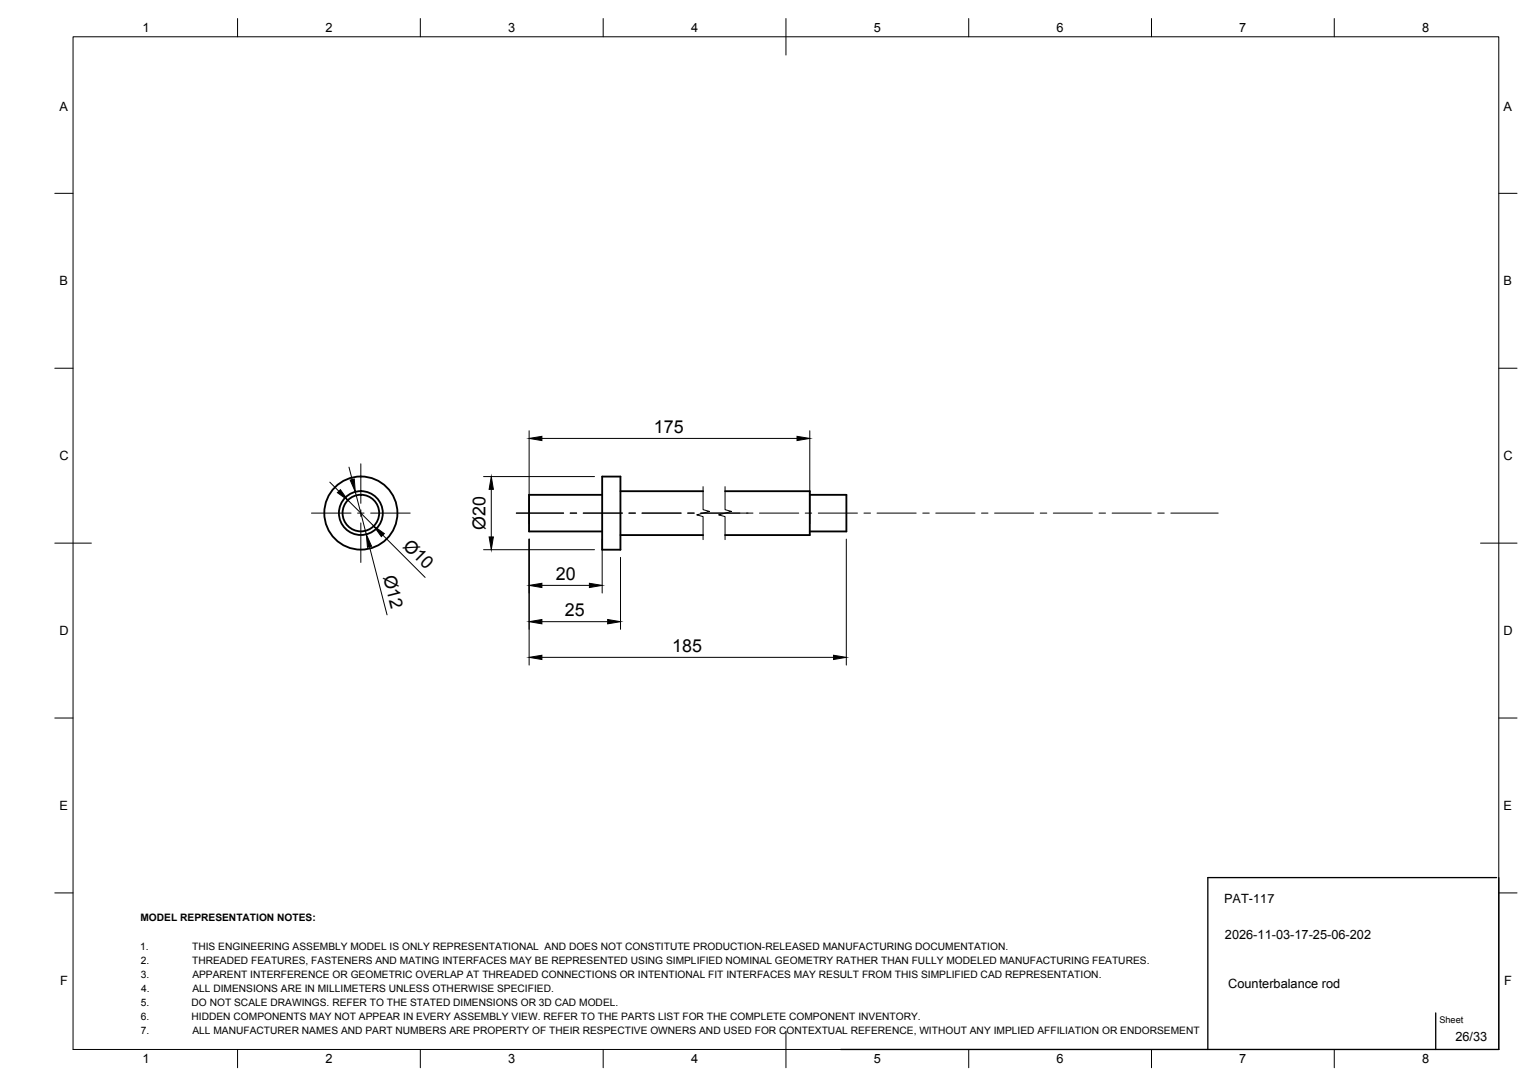
ISO-10303-21;
HEADER;
/* Generated by software containing ST-Developer
 * from STEP Tools, Inc. (www.steptools.com) 
 */

FILE_DESCRIPTION(
/* description */ ('Counterbalanced vertical column'),
/* implementation_level */ '2;1');

FILE_NAME(
/* name */ 'Counterbalance rod.step',
/* time_stamp */ '2026-10-29T16:47:22-07:00',
/* author */ (''),
/* organization */ (''),
/* preprocessor_version */ 'ST-DEVELOPER v20.2',
/* originating_system */ 'Autodesk Translation Framework v15.17.0.0',
/* authorisation */ '');

FILE_SCHEMA (('AUTOMOTIVE_DESIGN { 1 0 10303 214 3 1 1 }'));
ENDSEC;

DATA;
#10=MECHANICAL_DESIGN_GEOMETRIC_PRESENTATION_REPRESENTATION('',(#375),#15040);
#305=SHAPE_REPRESENTATION_RELATIONSHIP('SRR','None',#15210,#340);
#340=ADVANCED_BREP_SHAPE_REPRESENTATION('',(#408),#15029);
#375=STYLED_ITEM('',(#15457),#408);
#408=MANIFOLD_SOLID_BREP('Body1',#7100);
#516=FACE_BOUND('',#1633,.T.);
#517=FACE_BOUND('',#1636,.T.);
#518=FACE_BOUND('',#1639,.T.);
#743=PLANE('',#7996);
#744=PLANE('',#8000);
#745=PLANE('',#8001);
#746=PLANE('',#8006);
#747=PLANE('',#8009);
#1123=FACE_OUTER_BOUND('',#1628,.T.);
#1124=FACE_OUTER_BOUND('',#1629,.T.);
#1125=FACE_OUTER_BOUND('',#1630,.T.);
#1126=FACE_OUTER_BOUND('',#1631,.T.);
#1127=FACE_OUTER_BOUND('',#1632,.T.);
#1128=FACE_OUTER_BOUND('',#1634,.T.);
#1129=FACE_OUTER_BOUND('',#1635,.T.);
#1130=FACE_OUTER_BOUND('',#1637,.T.);
#1131=FACE_OUTER_BOUND('',#1638,.T.);
#1628=EDGE_LOOP('',(#6102,#6103,#6104,#6105));
#1629=EDGE_LOOP('',(#6106));
#1630=EDGE_LOOP('',(#6107,#6108,#6109,#6110));
#1631=EDGE_LOOP('',(#6111));
#1632=EDGE_LOOP('',(#6112));
#1633=EDGE_LOOP('',(#6113));
#1634=EDGE_LOOP('',(#6114,#6115,#6116,#6117));
#1635=EDGE_LOOP('',(#6118));
#1636=EDGE_LOOP('',(#6119));
#1637=EDGE_LOOP('',(#6120,#6121,#6122,#6123));
#1638=EDGE_LOOP('',(#6124));
#1639=EDGE_LOOP('',(#6125));
#2237=LINE('',#14397,#2908);
#2238=LINE('',#14404,#2909);
#2239=LINE('',#14415,#2910);
#2240=LINE('',#14419,#2911);
#2908=VECTOR('',#9701,0.5);
#2909=VECTOR('',#9710,0.5);
#2910=VECTOR('',#9725,1.);
#2911=VECTOR('',#9730,0.6);
#3255=CIRCLE('',#7994,0.5);
#3256=CIRCLE('',#7995,0.5);
#3257=CIRCLE('',#7998,0.5);
#3258=CIRCLE('',#7999,0.5);
#3259=CIRCLE('',#8002,1.);
#3260=CIRCLE('',#8003,0.6);
#3261=CIRCLE('',#8005,1.);
#3262=CIRCLE('',#8008,0.6);
#3740=VERTEX_POINT('',#14394);
#3741=VERTEX_POINT('',#14396);
#3742=VERTEX_POINT('',#14401);
#3743=VERTEX_POINT('',#14403);
#3744=VERTEX_POINT('',#14408);
#3745=VERTEX_POINT('',#14410);
#3746=VERTEX_POINT('',#14413);
#3747=VERTEX_POINT('',#14418);
#4552=EDGE_CURVE('',#3740,#3740,#3255,.T.);
#4553=EDGE_CURVE('',#3740,#3741,#2237,.T.);
#4554=EDGE_CURVE('',#3741,#3741,#3256,.T.);
#4555=EDGE_CURVE('',#3742,#3742,#3257,.T.);
#4556=EDGE_CURVE('',#3742,#3743,#2238,.T.);
#4557=EDGE_CURVE('',#3743,#3743,#3258,.T.);
#4558=EDGE_CURVE('',#3744,#3744,#3259,.T.);
#4559=EDGE_CURVE('',#3745,#3745,#3260,.T.);
#4560=EDGE_CURVE('',#3746,#3746,#3261,.T.);
#4561=EDGE_CURVE('',#3746,#3744,#2239,.T.);
#4562=EDGE_CURVE('',#3745,#3747,#2240,.T.);
#4563=EDGE_CURVE('',#3747,#3747,#3262,.T.);
#6102=ORIENTED_EDGE('',*,*,#4552,.F.);
#6103=ORIENTED_EDGE('',*,*,#4553,.T.);
#6104=ORIENTED_EDGE('',*,*,#4554,.F.);
#6105=ORIENTED_EDGE('',*,*,#4553,.F.);
#6106=ORIENTED_EDGE('',*,*,#4552,.T.);
#6107=ORIENTED_EDGE('',*,*,#4555,.F.);
#6108=ORIENTED_EDGE('',*,*,#4556,.T.);
#6109=ORIENTED_EDGE('',*,*,#4557,.T.);
#6110=ORIENTED_EDGE('',*,*,#4556,.F.);
#6111=ORIENTED_EDGE('',*,*,#4557,.F.);
#6112=ORIENTED_EDGE('',*,*,#4558,.F.);
#6113=ORIENTED_EDGE('',*,*,#4559,.T.);
#6114=ORIENTED_EDGE('',*,*,#4560,.F.);
#6115=ORIENTED_EDGE('',*,*,#4561,.T.);
#6116=ORIENTED_EDGE('',*,*,#4558,.T.);
#6117=ORIENTED_EDGE('',*,*,#4561,.F.);
#6118=ORIENTED_EDGE('',*,*,#4560,.T.);
#6119=ORIENTED_EDGE('',*,*,#4554,.T.);
#6120=ORIENTED_EDGE('',*,*,#4559,.F.);
#6121=ORIENTED_EDGE('',*,*,#4562,.T.);
#6122=ORIENTED_EDGE('',*,*,#4563,.T.);
#6123=ORIENTED_EDGE('',*,*,#4562,.F.);
#6124=ORIENTED_EDGE('',*,*,#4563,.F.);
#6125=ORIENTED_EDGE('',*,*,#4555,.T.);
#6650=CYLINDRICAL_SURFACE('',#7993,0.5);
#6651=CYLINDRICAL_SURFACE('',#7997,0.5);
#6652=CYLINDRICAL_SURFACE('',#8004,1.);
#6653=CYLINDRICAL_SURFACE('',#8007,0.6);
#6965=ADVANCED_FACE('',(#1123),#6650,.T.);
#6966=ADVANCED_FACE('',(#1124),#743,.T.);
#6967=ADVANCED_FACE('',(#1125),#6651,.T.);
#6968=ADVANCED_FACE('',(#1126),#744,.F.);
#6969=ADVANCED_FACE('',(#1127,#516),#745,.F.);
#6970=ADVANCED_FACE('',(#1128),#6652,.T.);
#6971=ADVANCED_FACE('',(#1129,#517),#746,.T.);
#6972=ADVANCED_FACE('',(#1130),#6653,.T.);
#6973=ADVANCED_FACE('',(#1131,#518),#747,.F.);
#7100=CLOSED_SHELL('',(#6965,#6966,#6967,#6968,#6969,#6970,#6971,#6972,
#6973));
#7992=AXIS2_PLACEMENT_3D('',#14392,#9695,#9696);
#7993=AXIS2_PLACEMENT_3D('',#14393,#9697,#9698);
#7994=AXIS2_PLACEMENT_3D('',#14395,#9699,#9700);
#7995=AXIS2_PLACEMENT_3D('',#14398,#9702,#9703);
#7996=AXIS2_PLACEMENT_3D('',#14399,#9704,#9705);
#7997=AXIS2_PLACEMENT_3D('',#14400,#9706,#9707);
#7998=AXIS2_PLACEMENT_3D('',#14402,#9708,#9709);
#7999=AXIS2_PLACEMENT_3D('',#14405,#9711,#9712);
#8000=AXIS2_PLACEMENT_3D('',#14406,#9713,#9714);
#8001=AXIS2_PLACEMENT_3D('',#14407,#9715,#9716);
#8002=AXIS2_PLACEMENT_3D('',#14409,#9717,#9718);
#8003=AXIS2_PLACEMENT_3D('',#14411,#9719,#9720);
#8004=AXIS2_PLACEMENT_3D('',#14412,#9721,#9722);
#8005=AXIS2_PLACEMENT_3D('',#14414,#9723,#9724);
#8006=AXIS2_PLACEMENT_3D('',#14416,#9726,#9727);
#8007=AXIS2_PLACEMENT_3D('',#14417,#9728,#9729);
#8008=AXIS2_PLACEMENT_3D('',#14420,#9731,#9732);
#8009=AXIS2_PLACEMENT_3D('',#14421,#9733,#9734);
#9695=DIRECTION('axis',(0.,0.,1.));
#9696=DIRECTION('refdir',(1.,0.,0.));
#9697=DIRECTION('center_axis',(0.,0.,1.));
#9698=DIRECTION('ref_axis',(1.,0.,0.));
#9699=DIRECTION('center_axis',(0.,0.,1.));
#9700=DIRECTION('ref_axis',(1.,0.,0.));
#9701=DIRECTION('',(0.,0.,-1.));
#9702=DIRECTION('center_axis',(0.,0.,-1.));
#9703=DIRECTION('ref_axis',(1.,0.,0.));
#9704=DIRECTION('center_axis',(0.,0.,1.));
#9705=DIRECTION('ref_axis',(1.,0.,0.));
#9706=DIRECTION('center_axis',(0.,0.,1.));
#9707=DIRECTION('ref_axis',(1.,0.,0.));
#9708=DIRECTION('center_axis',(0.,0.,1.));
#9709=DIRECTION('ref_axis',(1.,0.,0.));
#9710=DIRECTION('',(0.,0.,-1.));
#9711=DIRECTION('center_axis',(0.,0.,1.));
#9712=DIRECTION('ref_axis',(1.,0.,0.));
#9713=DIRECTION('center_axis',(0.,0.,1.));
#9714=DIRECTION('ref_axis',(1.,0.,0.));
#9715=DIRECTION('center_axis',(0.,0.,1.));
#9716=DIRECTION('ref_axis',(1.,0.,0.));
#9717=DIRECTION('center_axis',(0.,0.,1.));
#9718=DIRECTION('ref_axis',(1.,0.,0.));
#9719=DIRECTION('center_axis',(0.,0.,1.));
#9720=DIRECTION('ref_axis',(1.,0.,0.));
#9721=DIRECTION('center_axis',(0.,0.,1.));
#9722=DIRECTION('ref_axis',(1.,0.,0.));
#9723=DIRECTION('center_axis',(0.,0.,1.));
#9724=DIRECTION('ref_axis',(1.,0.,0.));
#9725=DIRECTION('',(0.,0.,-1.));
#9726=DIRECTION('center_axis',(0.,0.,1.));
#9727=DIRECTION('ref_axis',(1.,0.,0.));
#9728=DIRECTION('center_axis',(0.,0.,1.));
#9729=DIRECTION('ref_axis',(1.,0.,0.));
#9730=DIRECTION('',(0.,0.,-1.));
#9731=DIRECTION('center_axis',(0.,0.,1.));
#9732=DIRECTION('ref_axis',(1.,0.,0.));
#9733=DIRECTION('center_axis',(0.,0.,1.));
#9734=DIRECTION('ref_axis',(1.,0.,0.));
#14392=CARTESIAN_POINT('',(0.,0.,0.));
#14393=CARTESIAN_POINT('Origin',(-7.,0.,21.));
#14394=CARTESIAN_POINT('',(-7.5,-6.12323399573677E-17,23.));
#14395=CARTESIAN_POINT('Origin',(-7.,0.,23.));
#14396=CARTESIAN_POINT('',(-7.5,-6.12323399573677E-17,21.));
#14397=CARTESIAN_POINT('',(-7.5,-6.12323399573677E-17,21.));
#14398=CARTESIAN_POINT('Origin',(-7.,0.,21.));
#14399=CARTESIAN_POINT('Origin',(-7.,0.,23.));
#14400=CARTESIAN_POINT('Origin',(-7.,0.,4.5));
#14401=CARTESIAN_POINT('',(-7.5,-6.12323399573677E-17,5.5));
#14402=CARTESIAN_POINT('Origin',(-7.,0.,5.5));
#14403=CARTESIAN_POINT('',(-7.5,-6.12323399573677E-17,4.5));
#14404=CARTESIAN_POINT('',(-7.5,-6.12323399573677E-17,4.5));
#14405=CARTESIAN_POINT('Origin',(-7.,0.,4.5));
#14406=CARTESIAN_POINT('Origin',(-7.,0.,4.5));
#14407=CARTESIAN_POINT('Origin',(-7.,0.,20.5));
#14408=CARTESIAN_POINT('',(-8.,-1.22464679914735E-16,20.5));
#14409=CARTESIAN_POINT('Origin',(-7.,0.,20.5));
#14410=CARTESIAN_POINT('',(-7.6,-7.34788079488412E-17,20.5));
#14411=CARTESIAN_POINT('Origin',(-7.,0.,20.5));
#14412=CARTESIAN_POINT('Origin',(-7.,0.,20.5));
#14413=CARTESIAN_POINT('',(-8.,-1.22464679914735E-16,21.));
#14414=CARTESIAN_POINT('Origin',(-7.,0.,21.));
#14415=CARTESIAN_POINT('',(-8.,-1.22464679914735E-16,20.5));
#14416=CARTESIAN_POINT('Origin',(-7.,0.,21.));
#14417=CARTESIAN_POINT('Origin',(-7.,0.,5.5));
#14418=CARTESIAN_POINT('',(-7.6,-7.34788079488412E-17,5.5));
#14419=CARTESIAN_POINT('',(-7.6,-7.34788079488412E-17,5.5));
#14420=CARTESIAN_POINT('Origin',(-7.,0.,5.5));
#14421=CARTESIAN_POINT('Origin',(-7.,0.,5.5));
#14989=UNCERTAINTY_MEASURE_WITH_UNIT(LENGTH_MEASURE(0.001),#15041,
'DISTANCE_ACCURACY_VALUE',
'Maximum model space distance between geometric entities at asserted c
onnectivities');
#15000=UNCERTAINTY_MEASURE_WITH_UNIT(LENGTH_MEASURE(0.001),#15041,
'DISTANCE_ACCURACY_VALUE',
'Maximum model space distance between geometric entities at asserted c
onnectivities');
#15029=(
GEOMETRIC_REPRESENTATION_CONTEXT(3)
GLOBAL_UNCERTAINTY_ASSIGNED_CONTEXT((#14989))
GLOBAL_UNIT_ASSIGNED_CONTEXT((#15041,#15043,#15044))
REPRESENTATION_CONTEXT('','3D')
);
#15040=(
GEOMETRIC_REPRESENTATION_CONTEXT(3)
GLOBAL_UNCERTAINTY_ASSIGNED_CONTEXT((#15000))
GLOBAL_UNIT_ASSIGNED_CONTEXT((#15041,#15043,#15044))
REPRESENTATION_CONTEXT('','3D')
);
#15041=(
LENGTH_UNIT()
NAMED_UNIT(*)
SI_UNIT(.CENTI.,.METRE.)
);
#15043=(
NAMED_UNIT(*)
PLANE_ANGLE_UNIT()
SI_UNIT($,.RADIAN.)
);
#15044=(
NAMED_UNIT(*)
SI_UNIT($,.STERADIAN.)
SOLID_ANGLE_UNIT()
);
#15073=SHAPE_DEFINITION_REPRESENTATION(#15112,#15210);
#15112=PRODUCT_DEFINITION_SHAPE('',$,#15250);
#15210=SHAPE_REPRESENTATION('',(#7992),#15029);
#15221=PRODUCT_DEFINITION_CONTEXT('part definition',#15340,'design');
#15250=PRODUCT_DEFINITION('Counterbalance rod','Counterbalance rod',#15289,
#15221);
#15289=PRODUCT_DEFINITION_FORMATION('',$,#15370);
#15340=APPLICATION_CONTEXT(
'Core Data for Automotive Mechanical Design Process');
#15341=PRODUCT_CONTEXT('part definition',#15340,'mechanical');
#15370=PRODUCT('Counterbalance rod','Counterbalance rod',
'Counterbalance rod',(#15341));
#15451=COLOUR_RGB('Grey',0.48,0.52,0.57);
#15452=FILL_AREA_STYLE_COLOUR('',#15451);
#15453=FILL_AREA_STYLE('',(#15452));
#15454=SURFACE_STYLE_FILL_AREA(#15453);
#15455=SURFACE_SIDE_STYLE('',(#15454));
#15456=SURFACE_STYLE_USAGE(.BOTH.,#15455);
#15457=PRESENTATION_STYLE_ASSIGNMENT((#15456));
ENDSEC;
END-ISO-10303-21;
